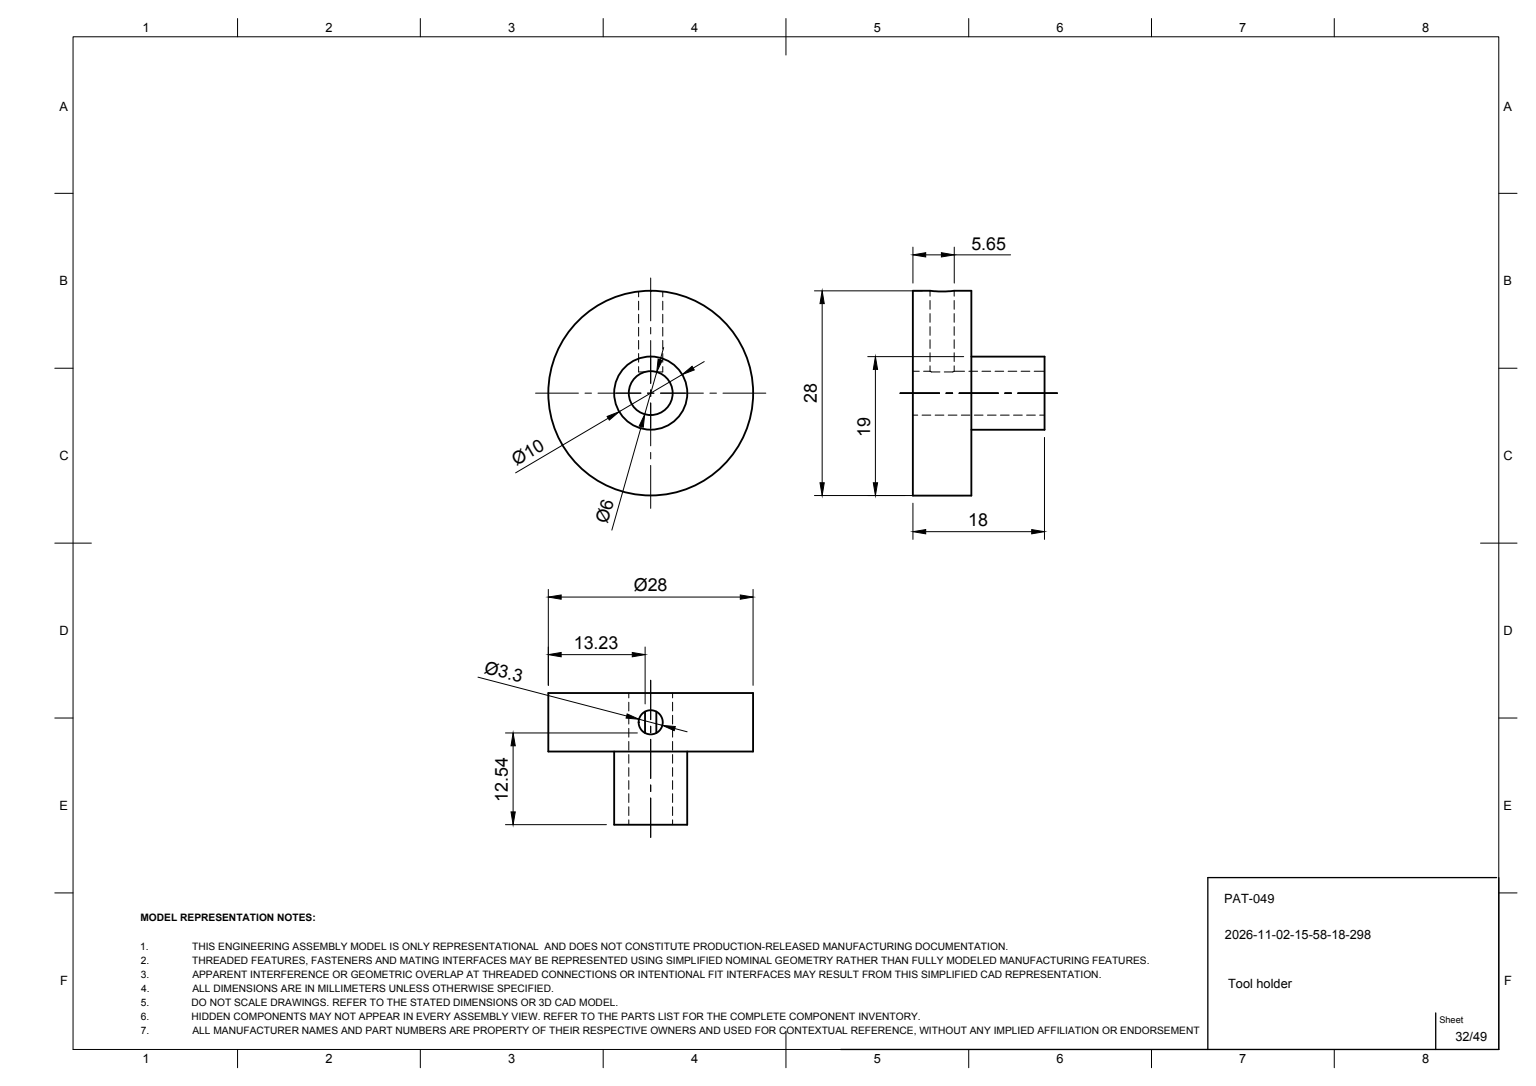
ISO-10303-21;
HEADER;
/* Generated by software containing ST-Developer
 * from STEP Tools, Inc. (www.steptools.com) 
 */

FILE_DESCRIPTION(
/* description */ ('Hand drill press frame (manual)'),
/* implementation_level */ '2;1');

FILE_NAME(
/* name */ 'Tool holder.step',
/* time_stamp */ '2026-10-28T03:25:28-07:00',
/* author */ (''),
/* organization */ (''),
/* preprocessor_version */ 'ST-DEVELOPER v20.2',
/* originating_system */ 'Autodesk Translation Framework v15.17.0.0',
/* authorisation */ '');

FILE_SCHEMA (('AUTOMOTIVE_DESIGN { 1 0 10303 214 3 1 1 }'));
ENDSEC;

DATA;
#10=MECHANICAL_DESIGN_GEOMETRIC_PRESENTATION_REPRESENTATION('',(#650),#33299);
#520=B_SPLINE_CURVE_WITH_KNOTS('',3,(#20783,#20784,#20785,#20786,#20787,
#20788,#20789,#20790,#20791,#20792),.UNSPECIFIED.,.F.,.F.,(4,2,2,2,4),(0.687371506923444,
0.701311490231616,0.76491921205255,0.828526933873483,0.842466917181656),
 .UNSPECIFIED.);
#521=B_SPLINE_CURVE_WITH_KNOTS('',3,(#20796,#20797,#20798,#20799,#20800,
#20801),.UNSPECIFIED.,.F.,.F.,(4,2,4),(0.254973070684183,0.318580792505117,
0.332520775813289),.UNSPECIFIED.);
#522=B_SPLINE_CURVE_WITH_KNOTS('',3,(#20805,#20806,#20807,#20808,#20809,
#20810,#20811,#20812,#20813,#20814,#20815,#20816,#20817,#20818,#20819,#20820,
#20821,#20822,#20823,#20824,#20825,#20826,#20827,#20828,#20829,#20830),
 .UNSPECIFIED.,.F.,.F.,(4,2,2,2,2,2,2,2,2,2,2,2,4),(0.,0.0622156192199746,
0.124431238439949,0.186646447577113,0.248861656714277,0.31107686585144,
0.373292074988604,0.435507694208578,0.497723313428553,0.559938932648528,
0.622154551868502,0.684369761005666,0.74658497014283),.UNSPECIFIED.);
#523=B_SPLINE_CURVE_WITH_KNOTS('',3,(#20831,#20832,#20833,#20834,#20835,
#20836,#20837,#20838,#20839,#20840),.UNSPECIFIED.,.F.,.F.,(4,2,2,2,4),(0.74658497014283,
0.808800179279993,0.871015388417157,0.933231007637132,0.995446626857106),
 .UNSPECIFIED.);
#524=B_SPLINE_CURVE_WITH_KNOTS('',3,(#20841,#20842,#20843,#20844,#20845,
#20846),.UNSPECIFIED.,.F.,.F.,(4,2,4),(0.177425365555079,0.19136534886325,
0.254973070684183),.UNSPECIFIED.);
#553=SHAPE_REPRESENTATION_RELATIONSHIP('SRR','None',#33514,#598);
#598=ADVANCED_BREP_SHAPE_REPRESENTATION('',(#701),#33276);
#650=STYLED_ITEM('',(#33807),#701);
#701=MANIFOLD_SOLID_BREP('Body1',#12669);
#847=FACE_BOUND('',#2612,.T.);
#848=FACE_BOUND('',#2615,.T.);
#849=FACE_BOUND('',#2617,.T.);
#850=FACE_BOUND('',#2619,.T.);
#851=FACE_BOUND('',#2621,.T.);
#1214=PLANE('',#13938);
#1215=PLANE('',#13942);
#1216=PLANE('',#13949);
#1217=PLANE('',#13953);
#1218=PLANE('',#13954);
#1792=FACE_OUTER_BOUND('',#2608,.T.);
#1793=FACE_OUTER_BOUND('',#2609,.T.);
#1794=FACE_OUTER_BOUND('',#2610,.T.);
#1795=FACE_OUTER_BOUND('',#2611,.T.);
#1796=FACE_OUTER_BOUND('',#2613,.T.);
#1797=FACE_OUTER_BOUND('',#2614,.T.);
#1798=FACE_OUTER_BOUND('',#2616,.T.);
#1799=FACE_OUTER_BOUND('',#2618,.T.);
#1800=FACE_OUTER_BOUND('',#2620,.T.);
#2608=EDGE_LOOP('',(#10719,#10720));
#2609=EDGE_LOOP('',(#10721,#10722,#10723,#10724,#10725,#10726,#10727,#10728,
#10729));
#2610=EDGE_LOOP('',(#10730,#10731));
#2611=EDGE_LOOP('',(#10732,#10733,#10734,#10735));
#2612=EDGE_LOOP('',(#10736,#10737,#10738,#10739,#10740));
#2613=EDGE_LOOP('',(#10741,#10742,#10743,#10744));
#2614=EDGE_LOOP('',(#10745));
#2615=EDGE_LOOP('',(#10746));
#2616=EDGE_LOOP('',(#10747,#10748,#10749,#10750));
#2617=EDGE_LOOP('',(#10751,#10752));
#2618=EDGE_LOOP('',(#10753));
#2619=EDGE_LOOP('',(#10754));
#2620=EDGE_LOOP('',(#10755));
#2621=EDGE_LOOP('',(#10756));
#3741=LINE('',#20779,#4906);
#3742=LINE('',#20803,#4907);
#3743=LINE('',#20848,#4908);
#3744=LINE('',#20853,#4909);
#3745=LINE('',#20859,#4910);
#3746=LINE('',#20866,#4911);
#4906=VECTOR('',#16726,1.);
#4907=VECTOR('',#16733,0.164999999999999);
#4908=VECTOR('',#16736,1.);
#4909=VECTOR('',#16741,0.3);
#4910=VECTOR('',#16748,0.5);
#4911=VECTOR('',#16757,1.4);
#5477=CIRCLE('',#13939,0.164999999999999);
#5478=CIRCLE('',#13941,0.164999999999999);
#5479=CIRCLE('',#13944,0.3);
#5480=CIRCLE('',#13945,0.3);
#5481=CIRCLE('',#13947,0.5);
#5482=CIRCLE('',#13948,0.5);
#5483=CIRCLE('',#13951,1.4);
#5484=CIRCLE('',#13952,1.4);
#6386=VERTEX_POINT('',#20777);
#6387=VERTEX_POINT('',#20778);
#6388=VERTEX_POINT('',#20782);
#6389=VERTEX_POINT('',#20793);
#6390=VERTEX_POINT('',#20795);
#6391=VERTEX_POINT('',#20802);
#6392=VERTEX_POINT('',#20804);
#6393=VERTEX_POINT('',#20850);
#6394=VERTEX_POINT('',#20852);
#6395=VERTEX_POINT('',#20856);
#6396=VERTEX_POINT('',#20858);
#6397=VERTEX_POINT('',#20863);
#6398=VERTEX_POINT('',#20865);
#7888=EDGE_CURVE('',#6386,#6387,#3741,.T.);
#7889=EDGE_CURVE('',#6386,#6387,#5477,.T.);
#7890=EDGE_CURVE('',#6388,#6386,#520,.T.);
#7891=EDGE_CURVE('',#6389,#6388,#5478,.T.);
#7892=EDGE_CURVE('',#6390,#6389,#521,.T.);
#7893=EDGE_CURVE('',#6390,#6391,#3742,.T.);
#7894=EDGE_CURVE('',#6392,#6391,#522,.T.);
#7895=EDGE_CURVE('',#6391,#6392,#523,.T.);
#7896=EDGE_CURVE('',#6387,#6390,#524,.T.);
#7897=EDGE_CURVE('',#6389,#6388,#3743,.T.);
#7898=EDGE_CURVE('',#6393,#6393,#5479,.T.);
#7899=EDGE_CURVE('',#6393,#6394,#3744,.T.);
#7900=EDGE_CURVE('',#6394,#6394,#5480,.T.);
#7901=EDGE_CURVE('',#6395,#6395,#5481,.T.);
#7902=EDGE_CURVE('',#6395,#6396,#3745,.T.);
#7903=EDGE_CURVE('',#6396,#6396,#5482,.T.);
#7904=EDGE_CURVE('',#6397,#6397,#5483,.T.);
#7905=EDGE_CURVE('',#6397,#6398,#3746,.T.);
#7906=EDGE_CURVE('',#6398,#6398,#5484,.T.);
#10719=ORIENTED_EDGE('',*,*,#7888,.F.);
#10720=ORIENTED_EDGE('',*,*,#7889,.T.);
#10721=ORIENTED_EDGE('',*,*,#7890,.F.);
#10722=ORIENTED_EDGE('',*,*,#7891,.F.);
#10723=ORIENTED_EDGE('',*,*,#7892,.F.);
#10724=ORIENTED_EDGE('',*,*,#7893,.T.);
#10725=ORIENTED_EDGE('',*,*,#7894,.F.);
#10726=ORIENTED_EDGE('',*,*,#7895,.F.);
#10727=ORIENTED_EDGE('',*,*,#7893,.F.);
#10728=ORIENTED_EDGE('',*,*,#7896,.F.);
#10729=ORIENTED_EDGE('',*,*,#7889,.F.);
#10730=ORIENTED_EDGE('',*,*,#7897,.F.);
#10731=ORIENTED_EDGE('',*,*,#7891,.T.);
#10732=ORIENTED_EDGE('',*,*,#7898,.F.);
#10733=ORIENTED_EDGE('',*,*,#7899,.T.);
#10734=ORIENTED_EDGE('',*,*,#7900,.F.);
#10735=ORIENTED_EDGE('',*,*,#7899,.F.);
#10736=ORIENTED_EDGE('',*,*,#7896,.T.);
#10737=ORIENTED_EDGE('',*,*,#7892,.T.);
#10738=ORIENTED_EDGE('',*,*,#7897,.T.);
#10739=ORIENTED_EDGE('',*,*,#7890,.T.);
#10740=ORIENTED_EDGE('',*,*,#7888,.T.);
#10741=ORIENTED_EDGE('',*,*,#7901,.F.);
#10742=ORIENTED_EDGE('',*,*,#7902,.T.);
#10743=ORIENTED_EDGE('',*,*,#7903,.F.);
#10744=ORIENTED_EDGE('',*,*,#7902,.F.);
#10745=ORIENTED_EDGE('',*,*,#7901,.T.);
#10746=ORIENTED_EDGE('',*,*,#7900,.T.);
#10747=ORIENTED_EDGE('',*,*,#7904,.F.);
#10748=ORIENTED_EDGE('',*,*,#7905,.T.);
#10749=ORIENTED_EDGE('',*,*,#7906,.T.);
#10750=ORIENTED_EDGE('',*,*,#7905,.F.);
#10751=ORIENTED_EDGE('',*,*,#7894,.T.);
#10752=ORIENTED_EDGE('',*,*,#7895,.T.);
#10753=ORIENTED_EDGE('',*,*,#7904,.T.);
#10754=ORIENTED_EDGE('',*,*,#7903,.T.);
#10755=ORIENTED_EDGE('',*,*,#7906,.F.);
#10756=ORIENTED_EDGE('',*,*,#7898,.T.);
#11887=CYLINDRICAL_SURFACE('',#13940,0.164999999999999);
#11888=CYLINDRICAL_SURFACE('',#13943,0.3);
#11889=CYLINDRICAL_SURFACE('',#13946,0.5);
#11890=CYLINDRICAL_SURFACE('',#13950,1.4);
#12401=ADVANCED_FACE('',(#1792),#1214,.T.);
#12402=ADVANCED_FACE('',(#1793),#11887,.F.);
#12403=ADVANCED_FACE('',(#1794),#1215,.T.);
#12404=ADVANCED_FACE('',(#1795,#847),#11888,.F.);
#12405=ADVANCED_FACE('',(#1796),#11889,.T.);
#12406=ADVANCED_FACE('',(#1797,#848),#1216,.T.);
#12407=ADVANCED_FACE('',(#1798,#849),#11890,.T.);
#12408=ADVANCED_FACE('',(#1799,#850),#1217,.T.);
#12409=ADVANCED_FACE('',(#1800,#851),#1218,.F.);
#12669=CLOSED_SHELL('',(#12401,#12402,#12403,#12404,#12405,#12406,#12407,
#12408,#12409));
#13937=AXIS2_PLACEMENT_3D('',#20775,#16722,#16723);
#13938=AXIS2_PLACEMENT_3D('',#20776,#16724,#16725);
#13939=AXIS2_PLACEMENT_3D('',#20780,#16727,#16728);
#13940=AXIS2_PLACEMENT_3D('',#20781,#16729,#16730);
#13941=AXIS2_PLACEMENT_3D('',#20794,#16731,#16732);
#13942=AXIS2_PLACEMENT_3D('',#20847,#16734,#16735);
#13943=AXIS2_PLACEMENT_3D('',#20849,#16737,#16738);
#13944=AXIS2_PLACEMENT_3D('',#20851,#16739,#16740);
#13945=AXIS2_PLACEMENT_3D('',#20854,#16742,#16743);
#13946=AXIS2_PLACEMENT_3D('',#20855,#16744,#16745);
#13947=AXIS2_PLACEMENT_3D('',#20857,#16746,#16747);
#13948=AXIS2_PLACEMENT_3D('',#20860,#16749,#16750);
#13949=AXIS2_PLACEMENT_3D('',#20861,#16751,#16752);
#13950=AXIS2_PLACEMENT_3D('',#20862,#16753,#16754);
#13951=AXIS2_PLACEMENT_3D('',#20864,#16755,#16756);
#13952=AXIS2_PLACEMENT_3D('',#20867,#16758,#16759);
#13953=AXIS2_PLACEMENT_3D('',#20868,#16760,#16761);
#13954=AXIS2_PLACEMENT_3D('',#20869,#16762,#16763);
#16722=DIRECTION('axis',(0.,0.,1.));
#16723=DIRECTION('refdir',(1.,0.,0.));
#16724=DIRECTION('center_axis',(1.,0.,0.));
#16725=DIRECTION('ref_axis',(0.,0.,-1.));
#16726=DIRECTION('',(0.,0.,1.));
#16727=DIRECTION('center_axis',(1.,0.,0.));
#16728=DIRECTION('ref_axis',(0.,0.,-1.));
#16729=DIRECTION('center_axis',(1.,0.,0.));
#16730=DIRECTION('ref_axis',(0.,0.,-1.));
#16731=DIRECTION('center_axis',(1.,0.,0.));
#16732=DIRECTION('ref_axis',(0.,0.,-1.));
#16733=DIRECTION('',(1.,0.,0.));
#16734=DIRECTION('center_axis',(1.,0.,0.));
#16735=DIRECTION('ref_axis',(0.,0.,-1.));
#16736=DIRECTION('',(0.,0.,-1.));
#16737=DIRECTION('center_axis',(0.,0.,1.));
#16738=DIRECTION('ref_axis',(1.,0.,0.));
#16739=DIRECTION('center_axis',(0.,0.,1.));
#16740=DIRECTION('ref_axis',(1.,0.,0.));
#16741=DIRECTION('',(0.,0.,1.));
#16742=DIRECTION('center_axis',(0.,0.,-1.));
#16743=DIRECTION('ref_axis',(1.,0.,0.));
#16744=DIRECTION('center_axis',(0.,0.,1.));
#16745=DIRECTION('ref_axis',(1.,0.,0.));
#16746=DIRECTION('center_axis',(0.,0.,1.));
#16747=DIRECTION('ref_axis',(1.,0.,0.));
#16748=DIRECTION('',(0.,0.,-1.));
#16749=DIRECTION('center_axis',(0.,0.,-1.));
#16750=DIRECTION('ref_axis',(1.,0.,0.));
#16751=DIRECTION('center_axis',(0.,0.,1.));
#16752=DIRECTION('ref_axis',(1.,0.,0.));
#16753=DIRECTION('center_axis',(0.,0.,1.));
#16754=DIRECTION('ref_axis',(1.,0.,0.));
#16755=DIRECTION('center_axis',(0.,0.,1.));
#16756=DIRECTION('ref_axis',(1.,0.,0.));
#16757=DIRECTION('',(0.,0.,-1.));
#16758=DIRECTION('center_axis',(0.,0.,1.));
#16759=DIRECTION('ref_axis',(1.,0.,0.));
#16760=DIRECTION('center_axis',(0.,0.,1.));
#16761=DIRECTION('ref_axis',(1.,0.,0.));
#16762=DIRECTION('center_axis',(0.,0.,1.));
#16763=DIRECTION('ref_axis',(1.,0.,0.));
#20775=CARTESIAN_POINT('',(0.,0.,0.));
#20776=CARTESIAN_POINT('Origin',(1.29,0.,10.4));
#20777=CARTESIAN_POINT('',(1.29,0.0768114574786861,10.2539691813349));
#20778=CARTESIAN_POINT('',(1.29,0.0768114574786861,10.5460308186651));
#20779=CARTESIAN_POINT('',(1.29,0.0768114574786861,9.9));
#20780=CARTESIAN_POINT('Origin',(1.29,0.,10.4));
#20781=CARTESIAN_POINT('Origin',(1.29,0.,10.4));
#20782=CARTESIAN_POINT('',(1.29,-0.0768114574786861,10.2539691813349));
#20783=CARTESIAN_POINT('Ctrl Pts',(1.29,-0.0768114574786869,10.2539691813349));
#20784=CARTESIAN_POINT('Ctrl Pts',(1.29112130391241,-0.0725779987568773,
10.2517424038809));
#20785=CARTESIAN_POINT('Ctrl Pts',(1.29217403693718,-0.0682275444786245,
10.2496896532208));
#20786=CARTESIAN_POINT('Ctrl Pts',(1.29755094970157,-0.0435167473439239,
10.2393317115009));
#20787=CARTESIAN_POINT('Ctrl Pts',(1.3,-0.0212025739403112,10.235));
#20788=CARTESIAN_POINT('Ctrl Pts',(1.3,0.0212025739403112,10.235));
#20789=CARTESIAN_POINT('Ctrl Pts',(1.29755094970157,0.0435167473439239,
10.2393317115009));
#20790=CARTESIAN_POINT('Ctrl Pts',(1.29217403693718,0.0682275444786249,
10.2496896532208));
#20791=CARTESIAN_POINT('Ctrl Pts',(1.29112130391241,0.0725779987568771,
10.2517424038809));
#20792=CARTESIAN_POINT('Ctrl Pts',(1.29,0.0768114574786869,10.2539691813349));
#20793=CARTESIAN_POINT('',(1.29,-0.0768114574786861,10.5460308186651));
#20794=CARTESIAN_POINT('Origin',(1.29,0.,10.4));
#20795=CARTESIAN_POINT('',(1.3,-6.633889141012E-18,10.565));
#20796=CARTESIAN_POINT('Ctrl Pts',(1.3,3.46944695195361E-17,10.565));
#20797=CARTESIAN_POINT('Ctrl Pts',(1.3,-0.0212025739403111,10.565));
#20798=CARTESIAN_POINT('Ctrl Pts',(1.29755094970157,-0.043516747343924,
10.5606682884991));
#20799=CARTESIAN_POINT('Ctrl Pts',(1.29217403693718,-0.0682275444786246,
10.5503103467792));
#20800=CARTESIAN_POINT('Ctrl Pts',(1.29112130391241,-0.072577998756877,
10.5482575961191));
#20801=CARTESIAN_POINT('Ctrl Pts',(1.29,-0.0768114574786861,10.5460308186651));
#20802=CARTESIAN_POINT('',(2.4,-2.02066721859312E-17,10.565));
#20803=CARTESIAN_POINT('',(1.29,-2.02066721859312E-17,10.565));
#20804=CARTESIAN_POINT('',(2.3902427845524,0.164999999999999,10.4));
#20805=CARTESIAN_POINT('Ctrl Pts',(2.3902427845524,0.164999999999999,10.4));
#20806=CARTESIAN_POINT('Ctrl Pts',(2.3902427845524,0.164999999999999,10.37926146026));
#20807=CARTESIAN_POINT('Ctrl Pts',(2.39075468722975,0.160851447474558,10.3571538860416));
#20808=CARTESIAN_POINT('Ctrl Pts',(2.39259968365095,0.144006627864299,10.3165070705051));
#20809=CARTESIAN_POINT('Ctrl Pts',(2.39390570229761,0.131311408395221,10.2979661706037));
#20810=CARTESIAN_POINT('Ctrl Pts',(2.39635413416378,0.102033925885227,10.2686886880937));
#20811=CARTESIAN_POINT('Ctrl Pts',(2.39765618378145,0.0834929839417275,
10.2559933930893));
#20812=CARTESIAN_POINT('Ctrl Pts',(2.39949208802221,0.042846026446056,10.2391485178689));
#20813=CARTESIAN_POINT('Ctrl Pts',(2.4,0.0207384030457212,10.235));
#20814=CARTESIAN_POINT('Ctrl Pts',(2.4,-0.0207384030457212,10.235));
#20815=CARTESIAN_POINT('Ctrl Pts',(2.39949208802221,-0.042846026446056,
10.2391485178689));
#20816=CARTESIAN_POINT('Ctrl Pts',(2.39765618378145,-0.0834929839417275,
10.2559933930893));
#20817=CARTESIAN_POINT('Ctrl Pts',(2.39635413416378,-0.102033925885227,
10.2686886880937));
#20818=CARTESIAN_POINT('Ctrl Pts',(2.39390570229761,-0.131311408395221,
10.2979661706037));
#20819=CARTESIAN_POINT('Ctrl Pts',(2.39259968365095,-0.144006627864299,
10.3165070705051));
#20820=CARTESIAN_POINT('Ctrl Pts',(2.39075468722975,-0.160851447474558,
10.3571538860416));
#20821=CARTESIAN_POINT('Ctrl Pts',(2.3902427845524,-0.164999999999999,10.37926146026));
#20822=CARTESIAN_POINT('Ctrl Pts',(2.3902427845524,-0.164999999999999,10.42073853974));
#20823=CARTESIAN_POINT('Ctrl Pts',(2.39075468722975,-0.160851447474558,
10.4428461139584));
#20824=CARTESIAN_POINT('Ctrl Pts',(2.39259968365095,-0.144006627864299,
10.4834929294949));
#20825=CARTESIAN_POINT('Ctrl Pts',(2.39390570229761,-0.131311408395221,
10.5020338293963));
#20826=CARTESIAN_POINT('Ctrl Pts',(2.39635413416378,-0.102033925885227,
10.5313113119063));
#20827=CARTESIAN_POINT('Ctrl Pts',(2.39765618378145,-0.0834929839417275,
10.5440066069107));
#20828=CARTESIAN_POINT('Ctrl Pts',(2.39949208802221,-0.042846026446056,
10.5608514821311));
#20829=CARTESIAN_POINT('Ctrl Pts',(2.4,-0.0207384030457212,10.565));
#20830=CARTESIAN_POINT('Ctrl Pts',(2.4,-2.60208521396521E-17,10.565));
#20831=CARTESIAN_POINT('Ctrl Pts',(2.4,1.04083408558608E-16,10.565));
#20832=CARTESIAN_POINT('Ctrl Pts',(2.4,0.0207384030457213,10.565));
#20833=CARTESIAN_POINT('Ctrl Pts',(2.39949208802221,0.042846026446056,10.5608514821311));
#20834=CARTESIAN_POINT('Ctrl Pts',(2.39765618378145,0.0834929839417275,
10.5440066069107));
#20835=CARTESIAN_POINT('Ctrl Pts',(2.39635413416378,0.102033925885227,10.5313113119063));
#20836=CARTESIAN_POINT('Ctrl Pts',(2.39390570229761,0.131311408395221,10.5020338293963));
#20837=CARTESIAN_POINT('Ctrl Pts',(2.39259968365095,0.144006627864299,10.4834929294949));
#20838=CARTESIAN_POINT('Ctrl Pts',(2.39075468722975,0.160851447474558,10.4428461139584));
#20839=CARTESIAN_POINT('Ctrl Pts',(2.3902427845524,0.164999999999999,10.42073853974));
#20840=CARTESIAN_POINT('Ctrl Pts',(2.3902427845524,0.164999999999999,10.4));
#20841=CARTESIAN_POINT('Ctrl Pts',(1.29,0.0768114574786861,10.5460308186651));
#20842=CARTESIAN_POINT('Ctrl Pts',(1.29112130391241,0.0725779987568767,
10.5482575961191));
#20843=CARTESIAN_POINT('Ctrl Pts',(1.29217403693718,0.0682275444786243,
10.5503103467792));
#20844=CARTESIAN_POINT('Ctrl Pts',(1.29755094970157,0.0435167473439239,
10.5606682884991));
#20845=CARTESIAN_POINT('Ctrl Pts',(1.3,0.0212025739403111,10.565));
#20846=CARTESIAN_POINT('Ctrl Pts',(1.3,-4.16333634234434E-17,10.565));
#20847=CARTESIAN_POINT('Origin',(1.29,0.,10.4));
#20848=CARTESIAN_POINT('',(1.29,-0.0768114574786861,9.9));
#20849=CARTESIAN_POINT('Origin',(1.,0.,9.9));
#20850=CARTESIAN_POINT('',(0.7,-3.67394039744206E-17,10.));
#20851=CARTESIAN_POINT('Origin',(1.,0.,10.));
#20852=CARTESIAN_POINT('',(0.7,3.67394039744206E-17,11.8));
#20853=CARTESIAN_POINT('',(0.7,-3.67394039744206E-17,9.9));
#20854=CARTESIAN_POINT('Origin',(1.,0.,11.8));
#20855=CARTESIAN_POINT('Origin',(1.,0.,10.8));
#20856=CARTESIAN_POINT('',(0.5,-6.12323399573677E-17,11.8));
#20857=CARTESIAN_POINT('Origin',(1.,0.,11.8));
#20858=CARTESIAN_POINT('',(0.5,-6.12323399573677E-17,10.8));
#20859=CARTESIAN_POINT('',(0.5,-6.12323399573677E-17,10.8));
#20860=CARTESIAN_POINT('Origin',(1.,0.,10.8));
#20861=CARTESIAN_POINT('Origin',(1.,0.,11.8));
#20862=CARTESIAN_POINT('Origin',(1.,0.,10.));
#20863=CARTESIAN_POINT('',(-0.4,-1.71450551880629E-16,10.8));
#20864=CARTESIAN_POINT('Origin',(1.,0.,10.8));
#20865=CARTESIAN_POINT('',(-0.4,-1.71450551880629E-16,10.));
#20866=CARTESIAN_POINT('',(-0.4,-1.71450551880629E-16,10.));
#20867=CARTESIAN_POINT('Origin',(1.,0.,10.));
#20868=CARTESIAN_POINT('Origin',(1.,0.,10.8));
#20869=CARTESIAN_POINT('Origin',(1.,0.,10.));
#33224=UNCERTAINTY_MEASURE_WITH_UNIT(LENGTH_MEASURE(0.001),#33300,
'DISTANCE_ACCURACY_VALUE',
'Maximum model space distance between geometric entities at asserted c
onnectivities');
#33247=UNCERTAINTY_MEASURE_WITH_UNIT(LENGTH_MEASURE(0.001),#33300,
'DISTANCE_ACCURACY_VALUE',
'Maximum model space distance between geometric entities at asserted c
onnectivities');
#33276=(
GEOMETRIC_REPRESENTATION_CONTEXT(3)
GLOBAL_UNCERTAINTY_ASSIGNED_CONTEXT((#33224))
GLOBAL_UNIT_ASSIGNED_CONTEXT((#33300,#33302,#33303))
REPRESENTATION_CONTEXT('','3D')
);
#33299=(
GEOMETRIC_REPRESENTATION_CONTEXT(3)
GLOBAL_UNCERTAINTY_ASSIGNED_CONTEXT((#33247))
GLOBAL_UNIT_ASSIGNED_CONTEXT((#33300,#33302,#33303))
REPRESENTATION_CONTEXT('','3D')
);
#33300=(
LENGTH_UNIT()
NAMED_UNIT(*)
SI_UNIT(.CENTI.,.METRE.)
);
#33302=(
NAMED_UNIT(*)
PLANE_ANGLE_UNIT()
SI_UNIT($,.RADIAN.)
);
#33303=(
NAMED_UNIT(*)
SI_UNIT($,.STERADIAN.)
SOLID_ANGLE_UNIT()
);
#33332=SHAPE_DEFINITION_REPRESENTATION(#33388,#33514);
#33388=PRODUCT_DEFINITION_SHAPE('',$,#33566);
#33514=SHAPE_REPRESENTATION('',(#13937),#33276);
#33537=PRODUCT_DEFINITION_CONTEXT('part definition',#33692,'design');
#33566=PRODUCT_DEFINITION('Tool holder','Tool holder',#33617,#33537);
#33617=PRODUCT_DEFINITION_FORMATION('',$,#33722);
#33692=APPLICATION_CONTEXT(
'Core Data for Automotive Mechanical Design Process');
#33693=PRODUCT_CONTEXT('part definition',#33692,'mechanical');
#33722=PRODUCT('Tool holder','Tool holder','Tool holder',(#33693));
#33801=COLOUR_RGB('Sky Blue',0.24,0.69,0.87);
#33802=FILL_AREA_STYLE_COLOUR('',#33801);
#33803=FILL_AREA_STYLE('',(#33802));
#33804=SURFACE_STYLE_FILL_AREA(#33803);
#33805=SURFACE_SIDE_STYLE('',(#33804));
#33806=SURFACE_STYLE_USAGE(.BOTH.,#33805);
#33807=PRESENTATION_STYLE_ASSIGNMENT((#33806));
ENDSEC;
END-ISO-10303-21;
